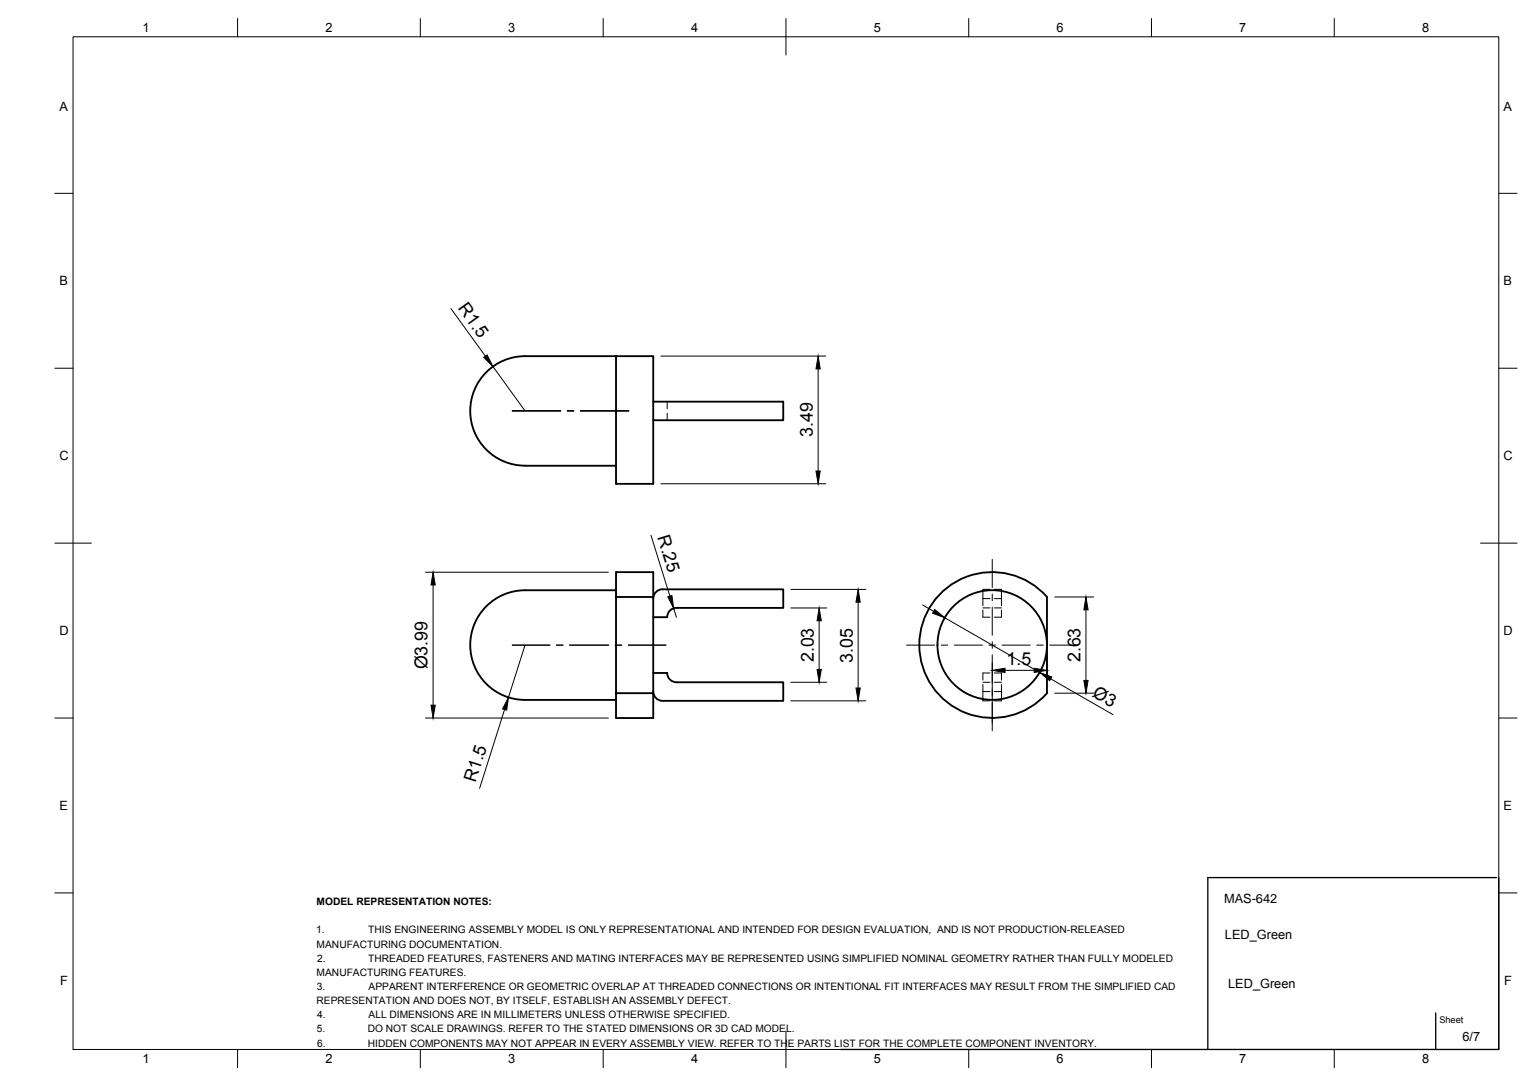
ISO-10303-21;
HEADER;
FILE_DESCRIPTION((''),'2;1');
FILE_NAME('LED_Green.step','2026-10-09T09:51:33-07:00',(''),(''),'','','');
FILE_SCHEMA (('AUTOMOTIVE_DESIGN { 1 0 10303 214 3 1 1 }'));
ENDSEC;
DATA;
#10=MECHANICAL_DESIGN_GEOMETRIC_PRESENTATION_REPRESENTATION('',(#1932,#1933,#1934,#1935,#1936,#1937,#1938),#126571);
#471=SHAPE_REPRESENTATION_RELATIONSHIP('SRR','None',#126601,#477) ;
#477=ADVANCED_BREP_SHAPE_REPRESENTATION('',(#4178),#126567) ;
#1932=STYLED_ITEM('',(#126643),#65340) ;
#1933=STYLED_ITEM('',(#126643),#65341) ;
#1934=STYLED_ITEM('',(#126643),#65356) ;
#1935=STYLED_ITEM('',(#126643),#65357) ;
#1936=STYLED_ITEM('',(#126643),#65358) ;
#1937=STYLED_ITEM('',(#126643),#65359) ;
#1938=STYLED_ITEM('',(#126642),#4178) ;
#4178=MANIFOLD_SOLID_BREP('Body1',#67692) ;
#4426=SPHERICAL_SURFACE('',#71862,1.4986) ;
#5029=FACE_BOUND('',#22354,.T.) ;
#5030=FACE_BOUND('',#22355,.T.) ;
#5468=PLANE('',#71837) ;
#5469=PLANE('',#71840) ;
#5470=PLANE('',#71843) ;
#5471=PLANE('',#71844) ;
#5472=PLANE('',#71847) ;
#5473=PLANE('',#71848) ;
#5474=PLANE('',#71851) ;
#5475=PLANE('',#71852) ;
#5476=PLANE('',#71853) ;
#5477=PLANE('',#71854) ;
#5478=PLANE('',#71859) ;
#5479=PLANE('',#71860) ;
#5480=PLANE('',#71861) ;
#5481=PLANE('',#71864) ;
#5482=PLANE('',#71865) ;
#6796=CYLINDRICAL_SURFACE('',#71830,1.4986) ;
#6797=CYLINDRICAL_SURFACE('',#71834,1.9939) ;
#6798=CYLINDRICAL_SURFACE('',#71855,0.254) ;
#6799=CYLINDRICAL_SURFACE('',#71856,0.254) ;
#6800=CYLINDRICAL_SURFACE('',#71857,0.254) ;
#6801=CYLINDRICAL_SURFACE('',#71858,0.254) ;
#9766=LINE('',#113750,#13882) ;
#9767=LINE('',#113759,#13883) ;
#9768=LINE('',#113762,#13884) ;
#9769=LINE('',#113768,#13885) ;
#9770=LINE('',#113770,#13886) ;
#9771=LINE('',#113774,#13887) ;
#9772=LINE('',#113776,#13888) ;
#9773=LINE('',#113777,#13889) ;
#9774=LINE('',#113781,#13890) ;
#9775=LINE('',#113783,#13891) ;
#9776=LINE('',#113787,#13892) ;
#9777=LINE('',#113789,#13893) ;
#9778=LINE('',#113791,#13894) ;
#9779=LINE('',#113794,#13895) ;
#9780=LINE('',#113795,#13896) ;
#9781=LINE('',#113799,#13897) ;
#9782=LINE('',#113801,#13898) ;
#9783=LINE('',#113805,#13899) ;
#9784=LINE('',#113807,#13900) ;
#9785=LINE('',#113809,#13901) ;
#9786=LINE('',#113814,#13902) ;
#9787=LINE('',#113815,#13903) ;
#9788=LINE('',#113816,#13904) ;
#9789=LINE('',#113822,#13905) ;
#9790=LINE('',#113824,#13906) ;
#9791=LINE('',#113827,#13907) ;
#9792=LINE('',#113828,#13908) ;
#9793=LINE('',#113830,#13909) ;
#9794=LINE('',#113831,#13910) ;
#9795=LINE('',#113834,#13911) ;
#9796=LINE('',#113835,#13912) ;
#9797=LINE('',#113838,#13913) ;
#9798=LINE('',#113840,#13914) ;
#9799=LINE('',#113842,#13915) ;
#9800=LINE('',#113844,#13916) ;
#9801=LINE('',#113846,#13917) ;
#9802=LINE('',#113847,#13918) ;
#9803=LINE('',#113848,#13919) ;
#9804=LINE('',#113850,#13920) ;
#9805=LINE('',#113851,#13921) ;
#13882=VECTOR('',#86860,1.4986) ;
#13883=VECTOR('',#86869,1000.) ;
#13884=VECTOR('',#86872,1000.) ;
#13885=VECTOR('',#86877,1000.) ;
#13886=VECTOR('',#86878,1000.) ;
#13887=VECTOR('',#86881,1000.) ;
#13888=VECTOR('',#86882,1000.) ;
#13889=VECTOR('',#86883,1000.) ;
#13890=VECTOR('',#86886,1000.) ;
#13891=VECTOR('',#86887,1000.) ;
#13892=VECTOR('',#86890,1000.) ;
#13893=VECTOR('',#86891,1000.) ;
#13894=VECTOR('',#86892,1000.) ;
#13895=VECTOR('',#86897,1000.) ;
#13896=VECTOR('',#86898,1000.) ;
#13897=VECTOR('',#86901,1000.) ;
#13898=VECTOR('',#86902,1000.) ;
#13899=VECTOR('',#86905,1000.) ;
#13900=VECTOR('',#86906,1000.) ;
#13901=VECTOR('',#86907,1000.) ;
#13902=VECTOR('',#86912,1000.) ;
#13903=VECTOR('',#86913,1000.) ;
#13904=VECTOR('',#86914,1000.) ;
#13905=VECTOR('',#86919,1000.) ;
#13906=VECTOR('',#86920,1000.) ;
#13907=VECTOR('',#86923,1000.) ;
#13908=VECTOR('',#86924,1000.) ;
#13909=VECTOR('',#86927,1000.) ;
#13910=VECTOR('',#86928,1000.) ;
#13911=VECTOR('',#86933,1000.) ;
#13912=VECTOR('',#86934,1000.) ;
#13913=VECTOR('',#86939,1000.) ;
#13914=VECTOR('',#86942,1000.) ;
#13915=VECTOR('',#86945,1000.) ;
#13916=VECTOR('',#86948,1000.) ;
#13917=VECTOR('',#86951,1000.) ;
#13918=VECTOR('',#86952,1000.) ;
#13919=VECTOR('',#86953,1000.) ;
#13920=VECTOR('',#86956,1000.) ;
#13921=VECTOR('',#86957,1000.) ;
#18055=FACE_OUTER_BOUND('',#22337,.T.) ;
#18056=FACE_OUTER_BOUND('',#22338,.T.) ;
#18057=FACE_OUTER_BOUND('',#22339,.T.) ;
#18058=FACE_OUTER_BOUND('',#22340,.T.) ;
#18059=FACE_OUTER_BOUND('',#22341,.T.) ;
#18060=FACE_OUTER_BOUND('',#22342,.T.) ;
#18061=FACE_OUTER_BOUND('',#22343,.T.) ;
#18062=FACE_OUTER_BOUND('',#22344,.T.) ;
#18063=FACE_OUTER_BOUND('',#22345,.T.) ;
#18064=FACE_OUTER_BOUND('',#22346,.T.) ;
#18065=FACE_OUTER_BOUND('',#22347,.T.) ;
#18066=FACE_OUTER_BOUND('',#22348,.T.) ;
#18067=FACE_OUTER_BOUND('',#22349,.T.) ;
#18068=FACE_OUTER_BOUND('',#22350,.T.) ;
#18069=FACE_OUTER_BOUND('',#22351,.T.) ;
#18070=FACE_OUTER_BOUND('',#22352,.T.) ;
#18071=FACE_OUTER_BOUND('',#22353,.T.) ;
#18072=FACE_OUTER_BOUND('',#22356,.T.) ;
#18073=FACE_OUTER_BOUND('',#22357,.T.) ;
#18074=FACE_OUTER_BOUND('',#22358,.T.) ;
#18075=FACE_OUTER_BOUND('',#22359,.T.) ;
#18076=FACE_OUTER_BOUND('',#22360,.T.) ;
#22337=EDGE_LOOP('',(#52750,#52751,#52752,#52753,#52754)) ;
#22338=EDGE_LOOP('',(#52755,#52756,#52757,#52758)) ;
#22339=EDGE_LOOP('',(#52759,#52760,#52761,#52762,#52763,#52764,#52765)) ;
#22340=EDGE_LOOP('',(#52766,#52767,#52768,#52769,#52770,#52771,#52772)) ;
#22341=EDGE_LOOP('',(#52773,#52774,#52775,#52776)) ;
#22342=EDGE_LOOP('',(#52777,#52778,#52779,#52780,#52781,#52782,#52783)) ;
#22343=EDGE_LOOP('',(#52784,#52785,#52786,#52787)) ;
#22344=EDGE_LOOP('',(#52788,#52789,#52790,#52791,#52792,#52793,#52794)) ;
#22345=EDGE_LOOP('',(#52795,#52796,#52797,#52798)) ;
#22346=EDGE_LOOP('',(#52799,#52800,#52801,#52802)) ;
#22347=EDGE_LOOP('',(#52803,#52804,#52805,#52806)) ;
#22348=EDGE_LOOP('',(#52807,#52808,#52809,#52810)) ;
#22349=EDGE_LOOP('',(#52811,#52812,#52813,#52814)) ;
#22350=EDGE_LOOP('',(#52815,#52816,#52817,#52818)) ;
#22351=EDGE_LOOP('',(#52819,#52820,#52821,#52822)) ;
#22352=EDGE_LOOP('',(#52823,#52824,#52825,#52826)) ;
#22353=EDGE_LOOP('',(#52827,#52828)) ;
#22354=EDGE_LOOP('',(#52829,#52830,#52831,#52832)) ;
#22355=EDGE_LOOP('',(#52833,#52834,#52835,#52836)) ;
#22356=EDGE_LOOP('',(#52837,#52838,#52839,#52840,#52841)) ;
#22357=EDGE_LOOP('',(#52842,#52843,#52844,#52845)) ;
#22358=EDGE_LOOP('',(#52846,#52847,#52848,#52849)) ;
#22359=EDGE_LOOP('',(#52850,#52851,#52852,#52853)) ;
#22360=EDGE_LOOP('',(#52854,#52855,#52856,#52857)) ;
#26843=CIRCLE('',#71831,1.4986) ;
#26844=CIRCLE('',#71832,1.4986) ;
#26845=CIRCLE('',#71833,1.4986) ;
#26846=CIRCLE('',#71835,1.9939) ;
#26847=CIRCLE('',#71836,1.9939) ;
#26848=CIRCLE('',#71838,0.254) ;
#26849=CIRCLE('',#71839,0.254) ;
#26850=CIRCLE('',#71841,0.254) ;
#26851=CIRCLE('',#71842,0.254) ;
#26852=CIRCLE('',#71845,0.254) ;
#26853=CIRCLE('',#71846,0.254) ;
#26854=CIRCLE('',#71849,0.254) ;
#26855=CIRCLE('',#71850,0.254) ;
#26856=CIRCLE('',#71863,1.4986) ;
#31962=VERTEX_POINT('',#113747) ;
#31963=VERTEX_POINT('',#113749) ;
#31964=VERTEX_POINT('',#113751) ;
#31965=VERTEX_POINT('',#113755) ;
#31966=VERTEX_POINT('',#113756) ;
#31967=VERTEX_POINT('',#113758) ;
#31968=VERTEX_POINT('',#113760) ;
#31969=VERTEX_POINT('',#113764) ;
#31970=VERTEX_POINT('',#113765) ;
#31971=VERTEX_POINT('',#113767) ;
#31972=VERTEX_POINT('',#113769) ;
#31973=VERTEX_POINT('',#113771) ;
#31974=VERTEX_POINT('',#113773) ;
#31975=VERTEX_POINT('',#113775) ;
#31976=VERTEX_POINT('',#113779) ;
#31977=VERTEX_POINT('',#113780) ;
#31978=VERTEX_POINT('',#113782) ;
#31979=VERTEX_POINT('',#113784) ;
#31980=VERTEX_POINT('',#113786) ;
#31981=VERTEX_POINT('',#113788) ;
#31982=VERTEX_POINT('',#113790) ;
#31983=VERTEX_POINT('',#113797) ;
#31984=VERTEX_POINT('',#113798) ;
#31985=VERTEX_POINT('',#113800) ;
#31986=VERTEX_POINT('',#113802) ;
#31987=VERTEX_POINT('',#113804) ;
#31988=VERTEX_POINT('',#113806) ;
#31989=VERTEX_POINT('',#113808) ;
#31990=VERTEX_POINT('',#113812) ;
#31991=VERTEX_POINT('',#113813) ;
#31992=VERTEX_POINT('',#113818) ;
#31993=VERTEX_POINT('',#113819) ;
#31994=VERTEX_POINT('',#113821) ;
#31995=VERTEX_POINT('',#113823) ;
#31996=VERTEX_POINT('',#113826) ;
#31997=VERTEX_POINT('',#113854) ;
#39034=EDGE_CURVE('',#31962,#31962,#26843,.T.) ;
#39035=EDGE_CURVE('',#31962,#31963,#9766,.T.) ;
#39036=EDGE_CURVE('',#31963,#31964,#26844,.T.) ;
#39037=EDGE_CURVE('',#31964,#31963,#26845,.T.) ;
#39038=EDGE_CURVE('',#31965,#31966,#26846,.T.) ;
#39039=EDGE_CURVE('',#31965,#31967,#9767,.T.) ;
#39040=EDGE_CURVE('',#31967,#31968,#26847,.T.) ;
#39041=EDGE_CURVE('',#31966,#31968,#9768,.T.) ;
#39042=EDGE_CURVE('',#31969,#31970,#26848,.T.) ;
#39043=EDGE_CURVE('',#31971,#31970,#9769,.T.) ;
#39044=EDGE_CURVE('',#31972,#31971,#9770,.T.) ;
#39045=EDGE_CURVE('',#31972,#31973,#26849,.T.) ;
#39046=EDGE_CURVE('',#31973,#31974,#9771,.T.) ;
#39047=EDGE_CURVE('',#31975,#31974,#9772,.T.) ;
#39048=EDGE_CURVE('',#31975,#31969,#9773,.T.) ;
#39049=EDGE_CURVE('',#31976,#31977,#9774,.T.) ;
#39050=EDGE_CURVE('',#31976,#31978,#9775,.T.) ;
#39051=EDGE_CURVE('',#31978,#31979,#26850,.T.) ;
#39052=EDGE_CURVE('',#31980,#31979,#9776,.T.) ;
#39053=EDGE_CURVE('',#31981,#31980,#9777,.T.) ;
#39054=EDGE_CURVE('',#31982,#31981,#9778,.T.) ;
#39055=EDGE_CURVE('',#31982,#31977,#26851,.T.) ;
#39056=EDGE_CURVE('',#31973,#31982,#9779,.T.) ;
#39057=EDGE_CURVE('',#31974,#31981,#9780,.T.) ;
#39058=EDGE_CURVE('',#31983,#31984,#9781,.T.) ;
#39059=EDGE_CURVE('',#31985,#31983,#9782,.T.) ;
#39060=EDGE_CURVE('',#31985,#31986,#26852,.T.) ;
#39061=EDGE_CURVE('',#31987,#31986,#9783,.T.) ;
#39062=EDGE_CURVE('',#31988,#31987,#9784,.T.) ;
#39063=EDGE_CURVE('',#31989,#31988,#9785,.T.) ;
#39064=EDGE_CURVE('',#31989,#31984,#26853,.T.) ;
#39065=EDGE_CURVE('',#31990,#31991,#9786,.T.) ;
#39066=EDGE_CURVE('',#31990,#31989,#9787,.T.) ;
#39067=EDGE_CURVE('',#31991,#31988,#9788,.T.) ;
#39068=EDGE_CURVE('',#31992,#31993,#26854,.T.) ;
#39069=EDGE_CURVE('',#31993,#31994,#9789,.T.) ;
#39070=EDGE_CURVE('',#31995,#31994,#9790,.T.) ;
#39071=EDGE_CURVE('',#31995,#31990,#26855,.T.) ;
#39072=EDGE_CURVE('',#31996,#31991,#9791,.T.) ;
#39073=EDGE_CURVE('',#31996,#31992,#9792,.T.) ;
#39074=EDGE_CURVE('',#31979,#31969,#9793,.T.) ;
#39075=EDGE_CURVE('',#31980,#31975,#9794,.T.) ;
#39076=EDGE_CURVE('',#31986,#31992,#9795,.T.) ;
#39077=EDGE_CURVE('',#31987,#31996,#9796,.T.) ;
#39078=EDGE_CURVE('',#31977,#31972,#9797,.T.) ;
#39079=EDGE_CURVE('',#31984,#31995,#9798,.T.) ;
#39080=EDGE_CURVE('',#31970,#31978,#9799,.T.) ;
#39081=EDGE_CURVE('',#31993,#31985,#9800,.T.) ;
#39082=EDGE_CURVE('',#31968,#31967,#9801,.T.) ;
#39083=EDGE_CURVE('',#31976,#31971,#9802,.T.) ;
#39084=EDGE_CURVE('',#31994,#31983,#9803,.T.) ;
#39085=EDGE_CURVE('',#31962,#31965,#9804,.T.) ;
#39086=EDGE_CURVE('',#31966,#31962,#9805,.T.) ;
#39087=EDGE_CURVE('',#31997,#31964,#26856,.T.) ;
#52750=ORIENTED_EDGE('',*,*,#39034,.T.) ;
#52751=ORIENTED_EDGE('',*,*,#39035,.T.) ;
#52752=ORIENTED_EDGE('',*,*,#39036,.T.) ;
#52753=ORIENTED_EDGE('',*,*,#39037,.T.) ;
#52754=ORIENTED_EDGE('',*,*,#39035,.F.) ;
#52755=ORIENTED_EDGE('',*,*,#39038,.F.) ;
#52756=ORIENTED_EDGE('',*,*,#39039,.T.) ;
#52757=ORIENTED_EDGE('',*,*,#39040,.T.) ;
#52758=ORIENTED_EDGE('',*,*,#39041,.F.) ;
#52759=ORIENTED_EDGE('',*,*,#39042,.T.) ;
#52760=ORIENTED_EDGE('',*,*,#39043,.F.) ;
#52761=ORIENTED_EDGE('',*,*,#39044,.F.) ;
#52762=ORIENTED_EDGE('',*,*,#39045,.T.) ;
#52763=ORIENTED_EDGE('',*,*,#39046,.T.) ;
#52764=ORIENTED_EDGE('',*,*,#39047,.F.) ;
#52765=ORIENTED_EDGE('',*,*,#39048,.T.) ;
#52766=ORIENTED_EDGE('',*,*,#39049,.F.) ;
#52767=ORIENTED_EDGE('',*,*,#39050,.T.) ;
#52768=ORIENTED_EDGE('',*,*,#39051,.T.) ;
#52769=ORIENTED_EDGE('',*,*,#39052,.F.) ;
#52770=ORIENTED_EDGE('',*,*,#39053,.F.) ;
#52771=ORIENTED_EDGE('',*,*,#39054,.F.) ;
#52772=ORIENTED_EDGE('',*,*,#39055,.T.) ;
#52773=ORIENTED_EDGE('',*,*,#39046,.F.) ;
#52774=ORIENTED_EDGE('',*,*,#39056,.T.) ;
#52775=ORIENTED_EDGE('',*,*,#39054,.T.) ;
#52776=ORIENTED_EDGE('',*,*,#39057,.F.) ;
#52777=ORIENTED_EDGE('',*,*,#39058,.F.) ;
#52778=ORIENTED_EDGE('',*,*,#39059,.F.) ;
#52779=ORIENTED_EDGE('',*,*,#39060,.T.) ;
#52780=ORIENTED_EDGE('',*,*,#39061,.F.) ;
#52781=ORIENTED_EDGE('',*,*,#39062,.F.) ;
#52782=ORIENTED_EDGE('',*,*,#39063,.F.) ;
#52783=ORIENTED_EDGE('',*,*,#39064,.T.) ;
#52784=ORIENTED_EDGE('',*,*,#39065,.F.) ;
#52785=ORIENTED_EDGE('',*,*,#39066,.T.) ;
#52786=ORIENTED_EDGE('',*,*,#39063,.T.) ;
#52787=ORIENTED_EDGE('',*,*,#39067,.F.) ;
#52788=ORIENTED_EDGE('',*,*,#39068,.T.) ;
#52789=ORIENTED_EDGE('',*,*,#39069,.T.) ;
#52790=ORIENTED_EDGE('',*,*,#39070,.F.) ;
#52791=ORIENTED_EDGE('',*,*,#39071,.T.) ;
#52792=ORIENTED_EDGE('',*,*,#39065,.T.) ;
#52793=ORIENTED_EDGE('',*,*,#39072,.F.) ;
#52794=ORIENTED_EDGE('',*,*,#39073,.T.) ;
#52795=ORIENTED_EDGE('',*,*,#39052,.T.) ;
#52796=ORIENTED_EDGE('',*,*,#39074,.T.) ;
#52797=ORIENTED_EDGE('',*,*,#39048,.F.) ;
#52798=ORIENTED_EDGE('',*,*,#39075,.F.) ;
#52799=ORIENTED_EDGE('',*,*,#39057,.T.) ;
#52800=ORIENTED_EDGE('',*,*,#39053,.T.) ;
#52801=ORIENTED_EDGE('',*,*,#39075,.T.) ;
#52802=ORIENTED_EDGE('',*,*,#39047,.T.) ;
#52803=ORIENTED_EDGE('',*,*,#39061,.T.) ;
#52804=ORIENTED_EDGE('',*,*,#39076,.T.) ;
#52805=ORIENTED_EDGE('',*,*,#39073,.F.) ;
#52806=ORIENTED_EDGE('',*,*,#39077,.F.) ;
#52807=ORIENTED_EDGE('',*,*,#39067,.T.) ;
#52808=ORIENTED_EDGE('',*,*,#39062,.T.) ;
#52809=ORIENTED_EDGE('',*,*,#39077,.T.) ;
#52810=ORIENTED_EDGE('',*,*,#39072,.T.) ;
#52811=ORIENTED_EDGE('',*,*,#39055,.F.) ;
#52812=ORIENTED_EDGE('',*,*,#39056,.F.) ;
#52813=ORIENTED_EDGE('',*,*,#39045,.F.) ;
#52814=ORIENTED_EDGE('',*,*,#39078,.F.) ;
#52815=ORIENTED_EDGE('',*,*,#39064,.F.) ;
#52816=ORIENTED_EDGE('',*,*,#39066,.F.) ;
#52817=ORIENTED_EDGE('',*,*,#39071,.F.) ;
#52818=ORIENTED_EDGE('',*,*,#39079,.F.) ;
#52819=ORIENTED_EDGE('',*,*,#39051,.F.) ;
#52820=ORIENTED_EDGE('',*,*,#39080,.F.) ;
#52821=ORIENTED_EDGE('',*,*,#39042,.F.) ;
#52822=ORIENTED_EDGE('',*,*,#39074,.F.) ;
#52823=ORIENTED_EDGE('',*,*,#39060,.F.) ;
#52824=ORIENTED_EDGE('',*,*,#39081,.F.) ;
#52825=ORIENTED_EDGE('',*,*,#39068,.F.) ;
#52826=ORIENTED_EDGE('',*,*,#39076,.F.) ;
#52827=ORIENTED_EDGE('',*,*,#39082,.F.) ;
#52828=ORIENTED_EDGE('',*,*,#39040,.F.) ;
#52829=ORIENTED_EDGE('',*,*,#39083,.F.) ;
#52830=ORIENTED_EDGE('',*,*,#39049,.T.) ;
#52831=ORIENTED_EDGE('',*,*,#39078,.T.) ;
#52832=ORIENTED_EDGE('',*,*,#39044,.T.) ;
#52833=ORIENTED_EDGE('',*,*,#39070,.T.) ;
#52834=ORIENTED_EDGE('',*,*,#39084,.T.) ;
#52835=ORIENTED_EDGE('',*,*,#39058,.T.) ;
#52836=ORIENTED_EDGE('',*,*,#39079,.T.) ;
#52837=ORIENTED_EDGE('',*,*,#39082,.T.) ;
#52838=ORIENTED_EDGE('',*,*,#39039,.F.) ;
#52839=ORIENTED_EDGE('',*,*,#39085,.F.) ;
#52840=ORIENTED_EDGE('',*,*,#39086,.F.) ;
#52841=ORIENTED_EDGE('',*,*,#39041,.T.) ;
#52842=ORIENTED_EDGE('',*,*,#39086,.T.) ;
#52843=ORIENTED_EDGE('',*,*,#39034,.F.) ;
#52844=ORIENTED_EDGE('',*,*,#39085,.T.) ;
#52845=ORIENTED_EDGE('',*,*,#39038,.T.) ;
#52846=ORIENTED_EDGE('',*,*,#39037,.F.) ;
#52847=ORIENTED_EDGE('',*,*,#39087,.F.) ;
#52848=ORIENTED_EDGE('',*,*,#39087,.T.) ;
#52849=ORIENTED_EDGE('',*,*,#39036,.F.) ;
#52850=ORIENTED_EDGE('',*,*,#39083,.T.) ;
#52851=ORIENTED_EDGE('',*,*,#39043,.T.) ;
#52852=ORIENTED_EDGE('',*,*,#39080,.T.) ;
#52853=ORIENTED_EDGE('',*,*,#39050,.F.) ;
#52854=ORIENTED_EDGE('',*,*,#39081,.T.) ;
#52855=ORIENTED_EDGE('',*,*,#39059,.T.) ;
#52856=ORIENTED_EDGE('',*,*,#39084,.F.) ;
#52857=ORIENTED_EDGE('',*,*,#39069,.F.) ;
#65340=ADVANCED_FACE('',(#18055),#6796,.T.) ;
#65341=ADVANCED_FACE('',(#18056),#6797,.T.) ;
#65342=ADVANCED_FACE('',(#18057),#5468,.F.) ;
#65343=ADVANCED_FACE('',(#18058),#5469,.F.) ;
#65344=ADVANCED_FACE('',(#18059),#5470,.F.) ;
#65345=ADVANCED_FACE('',(#18060),#5471,.F.) ;
#65346=ADVANCED_FACE('',(#18061),#5472,.F.) ;
#65347=ADVANCED_FACE('',(#18062),#5473,.F.) ;
#65348=ADVANCED_FACE('',(#18063),#5474,.F.) ;
#65349=ADVANCED_FACE('',(#18064),#5475,.T.) ;
#65350=ADVANCED_FACE('',(#18065),#5476,.F.) ;
#65351=ADVANCED_FACE('',(#18066),#5477,.F.) ;
#65352=ADVANCED_FACE('',(#18067),#6798,.T.) ;
#65353=ADVANCED_FACE('',(#18068),#6799,.T.) ;
#65354=ADVANCED_FACE('',(#18069),#6800,.F.) ;
#65355=ADVANCED_FACE('',(#18070),#6801,.F.) ;
#65356=ADVANCED_FACE('',(#18071,#5029,#5030),#5478,.F.) ;
#65357=ADVANCED_FACE('',(#18072),#5479,.F.) ;
#65358=ADVANCED_FACE('',(#18073),#5480,.T.) ;
#65359=ADVANCED_FACE('',(#18074),#4426,.T.) ;
#65360=ADVANCED_FACE('',(#18075),#5481,.F.) ;
#65361=ADVANCED_FACE('',(#18076),#5482,.F.) ;
#67692=CLOSED_SHELL('',(#65340,#65341,#65342,#65343,#65344,#65345,#65346,
#65347,#65348,#65349,#65350,#65351,#65352,#65353,#65354,#65355,#65356,#65357,
#65358,#65359,#65360,#65361)) ;
#71829=AXIS2_PLACEMENT_3D('',#113745,#86854,#86855) ;
#71830=AXIS2_PLACEMENT_3D('',#113746,#86856,#86857) ;
#71831=AXIS2_PLACEMENT_3D('',#113748,#86858,#86859) ;
#71832=AXIS2_PLACEMENT_3D('',#113752,#86861,#86862) ;
#71833=AXIS2_PLACEMENT_3D('',#113753,#86863,#86864) ;
#71834=AXIS2_PLACEMENT_3D('',#113754,#86865,#86866) ;
#71835=AXIS2_PLACEMENT_3D('',#113757,#86867,#86868) ;
#71836=AXIS2_PLACEMENT_3D('',#113761,#86870,#86871) ;
#71837=AXIS2_PLACEMENT_3D('',#113763,#86873,#86874) ;
#71838=AXIS2_PLACEMENT_3D('',#113766,#86875,#86876) ;
#71839=AXIS2_PLACEMENT_3D('',#113772,#86879,#86880) ;
#71840=AXIS2_PLACEMENT_3D('',#113778,#86884,#86885) ;
#71841=AXIS2_PLACEMENT_3D('',#113785,#86888,#86889) ;
#71842=AXIS2_PLACEMENT_3D('',#113792,#86893,#86894) ;
#71843=AXIS2_PLACEMENT_3D('',#113793,#86895,#86896) ;
#71844=AXIS2_PLACEMENT_3D('',#113796,#86899,#86900) ;
#71845=AXIS2_PLACEMENT_3D('',#113803,#86903,#86904) ;
#71846=AXIS2_PLACEMENT_3D('',#113810,#86908,#86909) ;
#71847=AXIS2_PLACEMENT_3D('',#113811,#86910,#86911) ;
#71848=AXIS2_PLACEMENT_3D('',#113817,#86915,#86916) ;
#71849=AXIS2_PLACEMENT_3D('',#113820,#86917,#86918) ;
#71850=AXIS2_PLACEMENT_3D('',#113825,#86921,#86922) ;
#71851=AXIS2_PLACEMENT_3D('',#113829,#86925,#86926) ;
#71852=AXIS2_PLACEMENT_3D('',#113832,#86929,#86930) ;
#71853=AXIS2_PLACEMENT_3D('',#113833,#86931,#86932) ;
#71854=AXIS2_PLACEMENT_3D('',#113836,#86935,#86936) ;
#71855=AXIS2_PLACEMENT_3D('',#113837,#86937,#86938) ;
#71856=AXIS2_PLACEMENT_3D('',#113839,#86940,#86941) ;
#71857=AXIS2_PLACEMENT_3D('',#113841,#86943,#86944) ;
#71858=AXIS2_PLACEMENT_3D('',#113843,#86946,#86947) ;
#71859=AXIS2_PLACEMENT_3D('',#113845,#86949,#86950) ;
#71860=AXIS2_PLACEMENT_3D('',#113849,#86954,#86955) ;
#71861=AXIS2_PLACEMENT_3D('',#113852,#86958,#86959) ;
#71862=AXIS2_PLACEMENT_3D('',#113853,#86960,#86961) ;
#71863=AXIS2_PLACEMENT_3D('',#113855,#86962,#86963) ;
#71864=AXIS2_PLACEMENT_3D('',#113856,#86964,#86965) ;
#71865=AXIS2_PLACEMENT_3D('',#113857,#86966,#86967) ;
#86854=DIRECTION('axis',(0.,0.,1.)) ;
#86855=DIRECTION('refdir',(1.,0.,0.)) ;
#86856=DIRECTION('center_axis',(0.,-1.,0.)) ;
#86857=DIRECTION('ref_axis',(0.,0.,-1.)) ;
#86858=DIRECTION('center_axis',(0.,1.,0.)) ;
#86859=DIRECTION('ref_axis',(0.,0.,1.)) ;
#86860=DIRECTION('',(0.,1.,0.)) ;
#86861=DIRECTION('center_axis',(0.,-1.,0.)) ;
#86862=DIRECTION('ref_axis',(0.,0.,-1.)) ;
#86863=DIRECTION('center_axis',(0.,-1.,0.)) ;
#86864=DIRECTION('ref_axis',(0.,0.,-1.)) ;
#86865=DIRECTION('center_axis',(0.,-1.,0.)) ;
#86866=DIRECTION('ref_axis',(0.,0.,-1.)) ;
#86867=DIRECTION('center_axis',(0.,1.,0.)) ;
#86868=DIRECTION('ref_axis',(0.,0.,1.)) ;
#86869=DIRECTION('',(0.,-1.,0.)) ;
#86870=DIRECTION('center_axis',(0.,1.,0.)) ;
#86871=DIRECTION('ref_axis',(0.,0.,1.)) ;
#86872=DIRECTION('',(0.,-1.,0.)) ;
#86873=DIRECTION('center_axis',(0.,0.,-1.)) ;
#86874=DIRECTION('ref_axis',(-1.,0.,0.)) ;
#86875=DIRECTION('center_axis',(0.,0.,-1.)) ;
#86876=DIRECTION('ref_axis',(-1.,0.,0.)) ;
#86877=DIRECTION('',(0.,-1.,0.)) ;
#86878=DIRECTION('',(1.,0.,0.)) ;
#86879=DIRECTION('center_axis',(0.,0.,1.)) ;
#86880=DIRECTION('ref_axis',(-1.,-1.81411780829267E-15,0.)) ;
#86881=DIRECTION('',(0.,-1.,0.)) ;
#86882=DIRECTION('',(-1.,0.,0.)) ;
#86883=DIRECTION('',(0.,1.,0.)) ;
#86884=DIRECTION('center_axis',(0.,0.,1.)) ;
#86885=DIRECTION('ref_axis',(1.,0.,0.)) ;
#86886=DIRECTION('',(-1.,0.,0.)) ;
#86887=DIRECTION('',(0.,-1.,0.)) ;
#86888=DIRECTION('center_axis',(0.,0.,1.)) ;
#86889=DIRECTION('ref_axis',(1.,0.,0.)) ;
#86890=DIRECTION('',(0.,1.,0.)) ;
#86891=DIRECTION('',(1.,0.,0.)) ;
#86892=DIRECTION('',(0.,-1.,0.)) ;
#86893=DIRECTION('center_axis',(0.,0.,-1.)) ;
#86894=DIRECTION('ref_axis',(1.,0.,0.)) ;
#86895=DIRECTION('center_axis',(1.,0.,-1.0671281225251E-16)) ;
#86896=DIRECTION('ref_axis',(-1.0671281225251E-16,0.,-1.)) ;
#86897=DIRECTION('',(-1.0671281225251E-16,0.,-1.)) ;
#86898=DIRECTION('',(0.,0.,-1.)) ;
#86899=DIRECTION('center_axis',(0.,0.,-1.)) ;
#86900=DIRECTION('ref_axis',(-1.,0.,0.)) ;
#86901=DIRECTION('',(1.,0.,0.)) ;
#86902=DIRECTION('',(0.,1.,0.)) ;
#86903=DIRECTION('center_axis',(0.,0.,-1.)) ;
#86904=DIRECTION('ref_axis',(-1.,0.,0.)) ;
#86905=DIRECTION('',(0.,1.,0.)) ;
#86906=DIRECTION('',(-1.,0.,-1.0671281225251E-16)) ;
#86907=DIRECTION('',(0.,-1.,0.)) ;
#86908=DIRECTION('center_axis',(0.,0.,1.)) ;
#86909=DIRECTION('ref_axis',(-1.,0.,0.)) ;
#86910=DIRECTION('center_axis',(-1.,0.,0.)) ;
#86911=DIRECTION('ref_axis',(0.,0.,1.)) ;
#86912=DIRECTION('',(0.,-1.,0.)) ;
#86913=DIRECTION('',(0.,0.,1.)) ;
#86914=DIRECTION('',(0.,0.,1.)) ;
#86915=DIRECTION('center_axis',(0.,0.,1.)) ;
#86916=DIRECTION('ref_axis',(1.,0.,0.)) ;
#86917=DIRECTION('center_axis',(0.,0.,1.)) ;
#86918=DIRECTION('ref_axis',(1.,0.,0.)) ;
#86919=DIRECTION('',(0.,1.,0.)) ;
#86920=DIRECTION('',(-1.,0.,0.)) ;
#86921=DIRECTION('center_axis',(0.,0.,-1.)) ;
#86922=DIRECTION('ref_axis',(1.,-1.81411780829268E-15,0.)) ;
#86923=DIRECTION('',(1.,0.,0.)) ;
#86924=DIRECTION('',(0.,1.,0.)) ;
#86925=DIRECTION('center_axis',(-1.,0.,-2.13425624505021E-16)) ;
#86926=DIRECTION('ref_axis',(-2.13425624505021E-16,0.,1.)) ;
#86927=DIRECTION('',(-2.13425624505021E-16,0.,1.)) ;
#86928=DIRECTION('',(-2.13425624505021E-16,0.,1.)) ;
#86929=DIRECTION('center_axis',(0.,-1.,0.)) ;
#86930=DIRECTION('ref_axis',(0.,0.,-1.)) ;
#86931=DIRECTION('center_axis',(1.,0.,0.)) ;
#86932=DIRECTION('ref_axis',(0.,0.,-1.)) ;
#86933=DIRECTION('',(0.,0.,-1.)) ;
#86934=DIRECTION('',(0.,0.,-1.)) ;
#86935=DIRECTION('center_axis',(0.,1.,0.)) ;
#86936=DIRECTION('ref_axis',(0.,0.,1.)) ;
#86937=DIRECTION('center_axis',(-1.0671281225251E-16,0.,-1.)) ;
#86938=DIRECTION('ref_axis',(-1.,0.,1.0671281225251E-16)) ;
#86939=DIRECTION('',(1.0671281225251E-16,0.,1.)) ;
#86940=DIRECTION('center_axis',(0.,0.,1.)) ;
#86941=DIRECTION('ref_axis',(1.,0.,0.)) ;
#86942=DIRECTION('',(0.,0.,-1.)) ;
#86943=DIRECTION('center_axis',(2.13425624505021E-16,0.,-1.)) ;
#86944=DIRECTION('ref_axis',(-1.,0.,-2.13425624505021E-16)) ;
#86945=DIRECTION('',(2.13425624505021E-16,0.,-1.)) ;
#86946=DIRECTION('center_axis',(0.,0.,1.)) ;
#86947=DIRECTION('ref_axis',(1.,0.,0.)) ;
#86948=DIRECTION('',(0.,0.,1.)) ;
#86949=DIRECTION('center_axis',(0.,1.,0.)) ;
#86950=DIRECTION('ref_axis',(0.,0.,1.)) ;
#86951=DIRECTION('',(1.,0.,0.)) ;
#86952=DIRECTION('',(0.,0.,1.)) ;
#86953=DIRECTION('',(0.,0.,1.)) ;
#86954=DIRECTION('center_axis',(0.,0.,-1.)) ;
#86955=DIRECTION('ref_axis',(-1.,0.,0.)) ;
#86956=DIRECTION('',(1.,0.,0.)) ;
#86957=DIRECTION('',(1.,0.,0.)) ;
#86958=DIRECTION('center_axis',(0.,1.,0.)) ;
#86959=DIRECTION('ref_axis',(0.,0.,1.)) ;
#86960=DIRECTION('center_axis',(0.,1.,0.)) ;
#86961=DIRECTION('ref_axis',(1.,0.,0.)) ;
#86962=DIRECTION('center_axis',(1.22464679914735E-16,0.,1.)) ;
#86963=DIRECTION('ref_axis',(-1.,0.,1.22464679914735E-16)) ;
#86964=DIRECTION('center_axis',(-1.,0.,0.)) ;
#86965=DIRECTION('ref_axis',(0.,0.,1.)) ;
#86966=DIRECTION('center_axis',(1.,0.,0.)) ;
#86967=DIRECTION('ref_axis',(0.,0.,-1.)) ;
#113745=CARTESIAN_POINT('',(0.,0.,0.)) ;
#113746=CARTESIAN_POINT('Origin',(1.27,5.3848,0.)) ;
#113747=CARTESIAN_POINT('',(1.27,1.397,1.4986)) ;
#113748=CARTESIAN_POINT('Origin',(1.27,1.397,0.)) ;
#113749=CARTESIAN_POINT('',(1.27,3.8862,1.4986)) ;
#113750=CARTESIAN_POINT('',(1.27,5.3848,1.4986)) ;
#113751=CARTESIAN_POINT('',(-0.2286,3.8862,1.83525569320222E-16)) ;
#113752=CARTESIAN_POINT('Origin',(1.27,3.8862,0.)) ;
#113753=CARTESIAN_POINT('Origin',(1.27,3.8862,0.)) ;
#113754=CARTESIAN_POINT('Origin',(1.27,1.397,0.)) ;
#113755=CARTESIAN_POINT('',(2.58523201375271,1.397,1.4986)) ;
#113756=CARTESIAN_POINT('',(-0.0452320137527065,1.397,1.4986)) ;
#113757=CARTESIAN_POINT('Origin',(1.27,1.397,0.)) ;
#113758=CARTESIAN_POINT('',(2.58523201375271,0.381,1.4986)) ;
#113759=CARTESIAN_POINT('',(2.58523201375271,1.397,1.4986)) ;
#113760=CARTESIAN_POINT('',(-0.0452320137527065,0.381,1.4986)) ;
#113761=CARTESIAN_POINT('Origin',(1.27,0.381,0.)) ;
#113762=CARTESIAN_POINT('',(-0.0452320137527065,1.397,1.4986)) ;
#113763=CARTESIAN_POINT('Origin',(-0.254,0.381,0.254)) ;
#113764=CARTESIAN_POINT('',(0.254,-0.254,0.254)) ;
#113765=CARTESIAN_POINT('',(0.508,0.,0.254)) ;
#113766=CARTESIAN_POINT('Origin',(0.508,-0.254,0.254)) ;
#113767=CARTESIAN_POINT('',(0.508,0.381,0.254)) ;
#113768=CARTESIAN_POINT('',(0.508,0.381,0.254)) ;
#113769=CARTESIAN_POINT('',(0.,0.381,0.254)) ;
#113770=CARTESIAN_POINT('',(-0.254,0.381,0.254)) ;
#113771=CARTESIAN_POINT('',(-0.254,0.127,0.254)) ;
#113772=CARTESIAN_POINT('Origin',(0.,0.127,0.254)) ;
#113773=CARTESIAN_POINT('',(-0.254,-3.175,0.254)) ;
#113774=CARTESIAN_POINT('',(-0.254,0.381,0.254)) ;
#113775=CARTESIAN_POINT('',(0.254,-3.175,0.254)) ;
#113776=CARTESIAN_POINT('',(-0.254,-3.175,0.254)) ;
#113777=CARTESIAN_POINT('',(0.254,-3.175,0.254)) ;
#113778=CARTESIAN_POINT('Origin',(-0.254,0.381,-0.254)) ;
#113779=CARTESIAN_POINT('',(0.508,0.381,-0.254)) ;
#113780=CARTESIAN_POINT('',(-5.42101086242752E-17,0.381,-0.254)) ;
#113781=CARTESIAN_POINT('',(-0.254,0.381,-0.254)) ;
#113782=CARTESIAN_POINT('',(0.508,0.,-0.254)) ;
#113783=CARTESIAN_POINT('',(0.508,0.381,-0.254)) ;
#113784=CARTESIAN_POINT('',(0.254,-0.254,-0.254)) ;
#113785=CARTESIAN_POINT('Origin',(0.508,-0.254,-0.254)) ;
#113786=CARTESIAN_POINT('',(0.254,-3.175,-0.254)) ;
#113787=CARTESIAN_POINT('',(0.254,-3.175,-0.254)) ;
#113788=CARTESIAN_POINT('',(-0.254,-3.175,-0.254)) ;
#113789=CARTESIAN_POINT('',(-0.254,-3.175,-0.254)) ;
#113790=CARTESIAN_POINT('',(-0.254,0.127,-0.254)) ;
#113791=CARTESIAN_POINT('',(-0.254,0.381,-0.254)) ;
#113792=CARTESIAN_POINT('Origin',(-5.42101086242752E-17,0.127,-0.254)) ;
#113793=CARTESIAN_POINT('Origin',(-0.254,0.381,-0.254)) ;
#113794=CARTESIAN_POINT('',(-0.254,0.127,-0.254)) ;
#113795=CARTESIAN_POINT('',(-0.254,-3.175,0.254)) ;
#113796=CARTESIAN_POINT('Origin',(-0.254,0.381,0.254)) ;
#113797=CARTESIAN_POINT('',(2.032,0.381,0.254)) ;
#113798=CARTESIAN_POINT('',(2.54,0.381,0.254)) ;
#113799=CARTESIAN_POINT('',(-0.254,0.381,0.254)) ;
#113800=CARTESIAN_POINT('',(2.032,0.,0.254)) ;
#113801=CARTESIAN_POINT('',(2.032,0.381,0.254)) ;
#113802=CARTESIAN_POINT('',(2.286,-0.254,0.254)) ;
#113803=CARTESIAN_POINT('Origin',(2.032,-0.254,0.254)) ;
#113804=CARTESIAN_POINT('',(2.286,-3.175,0.254)) ;
#113805=CARTESIAN_POINT('',(2.286,-3.175,0.254)) ;
#113806=CARTESIAN_POINT('',(2.794,-3.175,0.254)) ;
#113807=CARTESIAN_POINT('',(2.794,-3.175,0.254)) ;
#113808=CARTESIAN_POINT('',(2.794,0.127,0.254)) ;
#113809=CARTESIAN_POINT('',(2.794,0.381,0.254)) ;
#113810=CARTESIAN_POINT('Origin',(2.54,0.127,0.254)) ;
#113811=CARTESIAN_POINT('Origin',(2.794,0.381,-0.254)) ;
#113812=CARTESIAN_POINT('',(2.794,0.127,-0.254)) ;
#113813=CARTESIAN_POINT('',(2.794,-3.175,-0.254)) ;
#113814=CARTESIAN_POINT('',(2.794,0.381,-0.254)) ;
#113815=CARTESIAN_POINT('',(2.794,0.127,0.254)) ;
#113816=CARTESIAN_POINT('',(2.794,-3.175,0.254)) ;
#113817=CARTESIAN_POINT('Origin',(-0.254,0.381,-0.254)) ;
#113818=CARTESIAN_POINT('',(2.286,-0.254,-0.254)) ;
#113819=CARTESIAN_POINT('',(2.032,0.,-0.254)) ;
#113820=CARTESIAN_POINT('Origin',(2.032,-0.254,-0.254)) ;
#113821=CARTESIAN_POINT('',(2.032,0.381,-0.254)) ;
#113822=CARTESIAN_POINT('',(2.032,0.381,-0.254)) ;
#113823=CARTESIAN_POINT('',(2.54,0.381,-0.254)) ;
#113824=CARTESIAN_POINT('',(-0.254,0.381,-0.254)) ;
#113825=CARTESIAN_POINT('Origin',(2.54,0.127,-0.254)) ;
#113826=CARTESIAN_POINT('',(2.286,-3.175,-0.254)) ;
#113827=CARTESIAN_POINT('',(2.794,-3.175,-0.254)) ;
#113828=CARTESIAN_POINT('',(2.286,-3.175,-0.254)) ;
#113829=CARTESIAN_POINT('Origin',(0.254,-3.175,0.254)) ;
#113830=CARTESIAN_POINT('',(0.254,-0.254,0.254)) ;
#113831=CARTESIAN_POINT('',(0.254,-3.175,0.254)) ;
#113832=CARTESIAN_POINT('Origin',(-0.254,-3.175,-0.254)) ;
#113833=CARTESIAN_POINT('Origin',(2.286,-3.175,0.254)) ;
#113834=CARTESIAN_POINT('',(2.286,-0.254,-0.254)) ;
#113835=CARTESIAN_POINT('',(2.286,-3.175,0.254)) ;
#113836=CARTESIAN_POINT('Origin',(2.794,-3.175,-0.254)) ;
#113837=CARTESIAN_POINT('Origin',(0.,0.127,0.254)) ;
#113838=CARTESIAN_POINT('',(-2.89245657190524E-33,0.381,0.254)) ;
#113839=CARTESIAN_POINT('Origin',(2.54,0.127,0.254)) ;
#113840=CARTESIAN_POINT('',(2.54,0.381,-0.254)) ;
#113841=CARTESIAN_POINT('Origin',(0.508,-0.254,0.254)) ;
#113842=CARTESIAN_POINT('',(0.508,0.,-0.254)) ;
#113843=CARTESIAN_POINT('Origin',(2.032,-0.254,0.254)) ;
#113844=CARTESIAN_POINT('',(2.032,0.,0.254)) ;
#113845=CARTESIAN_POINT('Origin',(1.27,0.381,0.)) ;
#113846=CARTESIAN_POINT('',(2.58523201375271,0.381,1.4986)) ;
#113847=CARTESIAN_POINT('',(0.508,0.381,-1.9939)) ;
#113848=CARTESIAN_POINT('',(2.032,0.381,-1.9939)) ;
#113849=CARTESIAN_POINT('Origin',(2.58523201375271,1.397,1.4986)) ;
#113850=CARTESIAN_POINT('',(2.58523201375271,1.397,1.4986)) ;
#113851=CARTESIAN_POINT('',(2.58523201375271,1.397,1.4986)) ;
#113852=CARTESIAN_POINT('Origin',(1.27,1.397,0.)) ;
#113853=CARTESIAN_POINT('Origin',(1.27,3.8862,0.)) ;
#113854=CARTESIAN_POINT('',(1.27,5.3848,1.12377000514853E-32)) ;
#113855=CARTESIAN_POINT('Origin',(1.27,3.8862,0.)) ;
#113856=CARTESIAN_POINT('Origin',(0.508,0.381,-1.9939)) ;
#113857=CARTESIAN_POINT('Origin',(2.032,0.381,-1.9939)) ;
#126559=UNCERTAINTY_MEASURE_WITH_UNIT(LENGTH_MEASURE(0.01),#126572,
'DISTANCE_ACCURACY_VALUE',
'Maximum model space distance between geometric entities at asserted c
onnectivities') ;
#126563=UNCERTAINTY_MEASURE_WITH_UNIT(LENGTH_MEASURE(0.01),#126572,
'DISTANCE_ACCURACY_VALUE',
'Maximum model space distance between geometric entities at asserted c
onnectivities') ;
#126567=(
GEOMETRIC_REPRESENTATION_CONTEXT(3)
GLOBAL_UNCERTAINTY_ASSIGNED_CONTEXT((#126559))
GLOBAL_UNIT_ASSIGNED_CONTEXT((#126572,#126574,#126575))
REPRESENTATION_CONTEXT('','3D')
) ;
#126571=(
GEOMETRIC_REPRESENTATION_CONTEXT(3)
GLOBAL_UNCERTAINTY_ASSIGNED_CONTEXT((#126563))
GLOBAL_UNIT_ASSIGNED_CONTEXT((#126572,#126574,#126575))
REPRESENTATION_CONTEXT('','3D')
) ;
#126572=(
LENGTH_UNIT()
NAMED_UNIT(*)
SI_UNIT(.MILLI.,.METRE.)
) ;
#126574=(
NAMED_UNIT(*)
PLANE_ANGLE_UNIT()
SI_UNIT($,.RADIAN.)
) ;
#126575=(
NAMED_UNIT(*)
SI_UNIT($,.STERADIAN.)
SOLID_ANGLE_UNIT()
) ;
#126579=SHAPE_DEFINITION_REPRESENTATION(#126586,#126601) ;
#126586=PRODUCT_DEFINITION_SHAPE('',$,#126609) ;
#126601=SHAPE_REPRESENTATION('',(#71829),#126567) ;
#126605=PRODUCT_DEFINITION_CONTEXT('part definition',#126628,'design') ;
#126609=PRODUCT_DEFINITION('LED_Green','LED_Green',#126616,#126605) ;
#126616=PRODUCT_DEFINITION_FORMATION('',$,#126633) ;
#126628=APPLICATION_CONTEXT(
'Core Data for Automotive Mechanical Design Process') ;
#126629=PRODUCT_CONTEXT('part definition',#126628,'mechanical') ;
#126633=PRODUCT('LED_Green','LED_Green',$,(#126629)) ;
#126642=PRESENTATION_STYLE_ASSIGNMENT((#126651)) ;
#126643=PRESENTATION_STYLE_ASSIGNMENT((#126652)) ;
#126651=SURFACE_STYLE_USAGE(.BOTH.,#126660) ;
#126652=SURFACE_STYLE_USAGE(.BOTH.,#126661) ;
#126660=SURFACE_SIDE_STYLE('',(#126669)) ;
#126661=SURFACE_SIDE_STYLE('',(#126670)) ;
#126669=SURFACE_STYLE_FILL_AREA(#126678) ;
#126670=SURFACE_STYLE_FILL_AREA(#126679) ;
#126678=FILL_AREA_STYLE('Opaque(128,128,128)',(#126687)) ;
#126679=FILL_AREA_STYLE('Opaque(0,255,0)',(#126688)) ;
#126687=FILL_AREA_STYLE_COLOUR('Opaque(128,128,128)',#126696) ;
#126688=FILL_AREA_STYLE_COLOUR('Opaque(0,255,0)',#126697) ;
#126696=COLOUR_RGB('Opaque(128,128,128)', 0.09019608, 0.27058824, 0.51372549) ;
#126697=COLOUR_RGB('Opaque(0,255,0)', 0.08235294, 0.09019608, 0.10196078) ;
ENDSEC;
END-ISO-10303-21;
